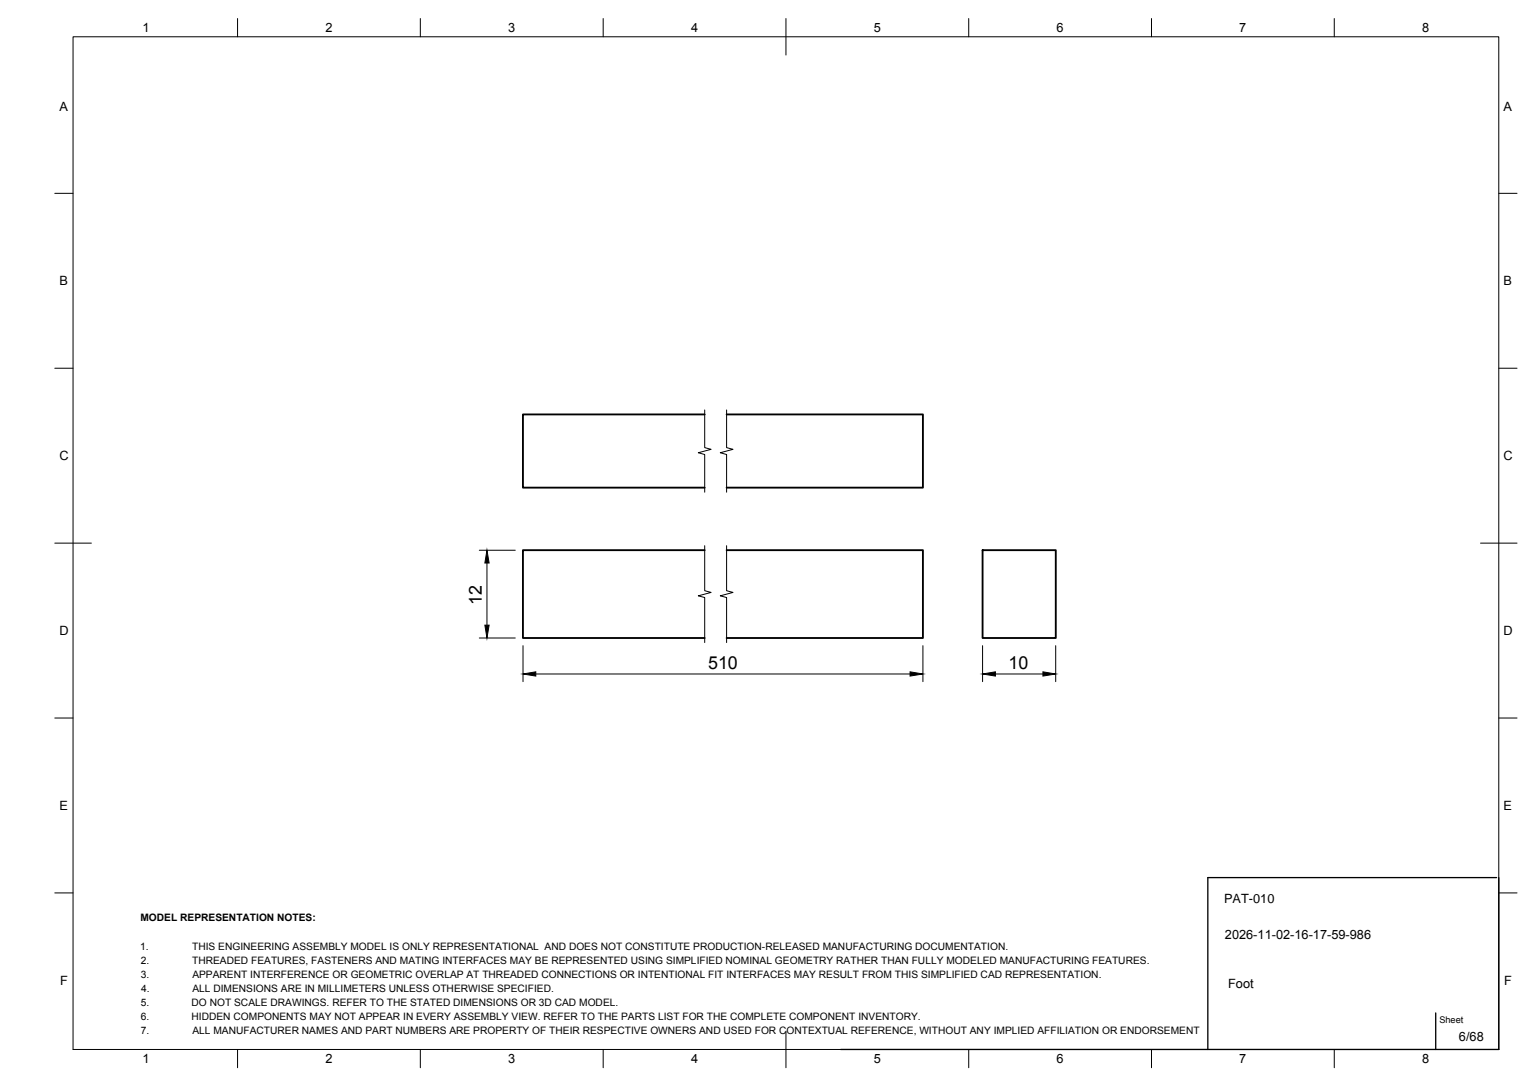
ISO-10303-21;
HEADER;
/* Generated by software containing ST-Developer
 * from STEP Tools, Inc. (www.steptools.com) 
 */

FILE_DESCRIPTION(
/* description */ ('Belt conveyor head drive unit'),
/* implementation_level */ '2;1');

FILE_NAME(
/* name */ 'Foot.step',
/* time_stamp */ '2026-10-28T03:26:19-07:00',
/* author */ (''),
/* organization */ (''),
/* preprocessor_version */ 'ST-DEVELOPER v20.2',
/* originating_system */ 'Autodesk Translation Framework v15.17.0.0',
/* authorisation */ '');

FILE_SCHEMA (('AUTOMOTIVE_DESIGN { 1 0 10303 214 3 1 1 }'));
ENDSEC;

DATA;
#10=MECHANICAL_DESIGN_GEOMETRIC_PRESENTATION_REPRESENTATION('',(#848),#27069);
#710=SHAPE_REPRESENTATION_RELATIONSHIP('SRR','None',#27354,#779);
#779=ADVANCED_BREP_SHAPE_REPRESENTATION('',(#933),#26996);
#848=STYLED_ITEM('',(#27811),#933);
#933=MANIFOLD_SOLID_BREP('Body1',#13713);
#1305=PLANE('',#14664);
#1306=PLANE('',#14665);
#1307=PLANE('',#14666);
#1308=PLANE('',#14667);
#1309=PLANE('',#14668);
#1310=PLANE('',#14669);
#1683=FACE_OUTER_BOUND('',#2503,.T.);
#1684=FACE_OUTER_BOUND('',#2504,.T.);
#1685=FACE_OUTER_BOUND('',#2505,.T.);
#1686=FACE_OUTER_BOUND('',#2506,.T.);
#1687=FACE_OUTER_BOUND('',#2507,.T.);
#1688=FACE_OUTER_BOUND('',#2508,.T.);
#2503=EDGE_LOOP('',(#9174,#9175,#9176,#9177));
#2504=EDGE_LOOP('',(#9178,#9179,#9180,#9181));
#2505=EDGE_LOOP('',(#9182,#9183,#9184,#9185));
#2506=EDGE_LOOP('',(#9186,#9187,#9188,#9189));
#2507=EDGE_LOOP('',(#9190,#9191,#9192,#9193));
#2508=EDGE_LOOP('',(#9194,#9195,#9196,#9197));
#3558=LINE('',#21207,#4350);
#3559=LINE('',#21209,#4351);
#3560=LINE('',#21211,#4352);
#3561=LINE('',#21212,#4353);
#3562=LINE('',#21215,#4354);
#3563=LINE('',#21217,#4355);
#3564=LINE('',#21218,#4356);
#3565=LINE('',#21221,#4357);
#3566=LINE('',#21223,#4358);
#3567=LINE('',#21224,#4359);
#3568=LINE('',#21226,#4360);
#3569=LINE('',#21227,#4361);
#4350=VECTOR('',#16700,1.);
#4351=VECTOR('',#16701,1.);
#4352=VECTOR('',#16702,1.);
#4353=VECTOR('',#16703,1.);
#4354=VECTOR('',#16706,1.);
#4355=VECTOR('',#16707,1.);
#4356=VECTOR('',#16708,1.);
#4357=VECTOR('',#16711,1.);
#4358=VECTOR('',#16712,1.);
#4359=VECTOR('',#16713,1.);
#4360=VECTOR('',#16716,1.);
#4361=VECTOR('',#16717,1.);
#6025=VERTEX_POINT('',#21205);
#6026=VERTEX_POINT('',#21206);
#6027=VERTEX_POINT('',#21208);
#6028=VERTEX_POINT('',#21210);
#6029=VERTEX_POINT('',#21214);
#6030=VERTEX_POINT('',#21216);
#6031=VERTEX_POINT('',#21220);
#6032=VERTEX_POINT('',#21222);
#7279=EDGE_CURVE('',#6025,#6026,#3558,.T.);
#7280=EDGE_CURVE('',#6026,#6027,#3559,.T.);
#7281=EDGE_CURVE('',#6028,#6027,#3560,.T.);
#7282=EDGE_CURVE('',#6025,#6028,#3561,.T.);
#7283=EDGE_CURVE('',#6029,#6025,#3562,.T.);
#7284=EDGE_CURVE('',#6030,#6028,#3563,.T.);
#7285=EDGE_CURVE('',#6029,#6030,#3564,.T.);
#7286=EDGE_CURVE('',#6031,#6029,#3565,.T.);
#7287=EDGE_CURVE('',#6032,#6030,#3566,.T.);
#7288=EDGE_CURVE('',#6031,#6032,#3567,.T.);
#7289=EDGE_CURVE('',#6026,#6031,#3568,.T.);
#7290=EDGE_CURVE('',#6027,#6032,#3569,.T.);
#9174=ORIENTED_EDGE('',*,*,#7279,.T.);
#9175=ORIENTED_EDGE('',*,*,#7280,.T.);
#9176=ORIENTED_EDGE('',*,*,#7281,.F.);
#9177=ORIENTED_EDGE('',*,*,#7282,.F.);
#9178=ORIENTED_EDGE('',*,*,#7283,.T.);
#9179=ORIENTED_EDGE('',*,*,#7282,.T.);
#9180=ORIENTED_EDGE('',*,*,#7284,.F.);
#9181=ORIENTED_EDGE('',*,*,#7285,.F.);
#9182=ORIENTED_EDGE('',*,*,#7286,.T.);
#9183=ORIENTED_EDGE('',*,*,#7285,.T.);
#9184=ORIENTED_EDGE('',*,*,#7287,.F.);
#9185=ORIENTED_EDGE('',*,*,#7288,.F.);
#9186=ORIENTED_EDGE('',*,*,#7289,.T.);
#9187=ORIENTED_EDGE('',*,*,#7288,.T.);
#9188=ORIENTED_EDGE('',*,*,#7290,.F.);
#9189=ORIENTED_EDGE('',*,*,#7280,.F.);
#9190=ORIENTED_EDGE('',*,*,#7290,.T.);
#9191=ORIENTED_EDGE('',*,*,#7287,.T.);
#9192=ORIENTED_EDGE('',*,*,#7284,.T.);
#9193=ORIENTED_EDGE('',*,*,#7281,.T.);
#9194=ORIENTED_EDGE('',*,*,#7289,.F.);
#9195=ORIENTED_EDGE('',*,*,#7279,.F.);
#9196=ORIENTED_EDGE('',*,*,#7283,.F.);
#9197=ORIENTED_EDGE('',*,*,#7286,.F.);
#12962=ADVANCED_FACE('',(#1683),#1305,.T.);
#12963=ADVANCED_FACE('',(#1684),#1306,.T.);
#12964=ADVANCED_FACE('',(#1685),#1307,.T.);
#12965=ADVANCED_FACE('',(#1686),#1308,.T.);
#12966=ADVANCED_FACE('',(#1687),#1309,.T.);
#12967=ADVANCED_FACE('',(#1688),#1310,.F.);
#13713=CLOSED_SHELL('',(#12962,#12963,#12964,#12965,#12966,#12967));
#14663=AXIS2_PLACEMENT_3D('',#21203,#16696,#16697);
#14664=AXIS2_PLACEMENT_3D('',#21204,#16698,#16699);
#14665=AXIS2_PLACEMENT_3D('',#21213,#16704,#16705);
#14666=AXIS2_PLACEMENT_3D('',#21219,#16709,#16710);
#14667=AXIS2_PLACEMENT_3D('',#21225,#16714,#16715);
#14668=AXIS2_PLACEMENT_3D('',#21228,#16718,#16719);
#14669=AXIS2_PLACEMENT_3D('',#21229,#16720,#16721);
#16696=DIRECTION('axis',(0.,0.,1.));
#16697=DIRECTION('refdir',(1.,0.,0.));
#16698=DIRECTION('center_axis',(0.,1.,0.));
#16699=DIRECTION('ref_axis',(-1.,0.,0.));
#16700=DIRECTION('',(-1.,0.,0.));
#16701=DIRECTION('',(0.,0.,1.));
#16702=DIRECTION('',(-1.,0.,0.));
#16703=DIRECTION('',(0.,0.,1.));
#16704=DIRECTION('center_axis',(1.,0.,0.));
#16705=DIRECTION('ref_axis',(0.,1.,0.));
#16706=DIRECTION('',(0.,1.,0.));
#16707=DIRECTION('',(0.,1.,0.));
#16708=DIRECTION('',(0.,0.,1.));
#16709=DIRECTION('center_axis',(0.,-1.,0.));
#16710=DIRECTION('ref_axis',(1.,0.,0.));
#16711=DIRECTION('',(1.,0.,0.));
#16712=DIRECTION('',(1.,0.,0.));
#16713=DIRECTION('',(0.,0.,1.));
#16714=DIRECTION('center_axis',(-1.,0.,0.));
#16715=DIRECTION('ref_axis',(0.,-1.,0.));
#16716=DIRECTION('',(0.,-1.,0.));
#16717=DIRECTION('',(0.,-1.,0.));
#16718=DIRECTION('center_axis',(0.,0.,1.));
#16719=DIRECTION('ref_axis',(1.,0.,0.));
#16720=DIRECTION('center_axis',(0.,0.,1.));
#16721=DIRECTION('ref_axis',(1.,0.,0.));
#21203=CARTESIAN_POINT('',(0.,0.,0.));
#21204=CARTESIAN_POINT('Origin',(-3.,44.5,-2.4));
#21205=CARTESIAN_POINT('',(-3.,44.5,-2.4));
#21206=CARTESIAN_POINT('',(-4.,44.5,-2.4));
#21207=CARTESIAN_POINT('',(-3.,44.5,-2.4));
#21208=CARTESIAN_POINT('',(-4.,44.5,-1.2));
#21209=CARTESIAN_POINT('',(-4.,44.5,-2.4));
#21210=CARTESIAN_POINT('',(-3.,44.5,-1.2));
#21211=CARTESIAN_POINT('',(-3.,44.5,-1.2));
#21212=CARTESIAN_POINT('',(-3.,44.5,-2.4));
#21213=CARTESIAN_POINT('Origin',(-3.,-6.5,-2.4));
#21214=CARTESIAN_POINT('',(-3.,-6.5,-2.4));
#21215=CARTESIAN_POINT('',(-3.,-6.5,-2.4));
#21216=CARTESIAN_POINT('',(-3.,-6.5,-1.2));
#21217=CARTESIAN_POINT('',(-3.,-6.5,-1.2));
#21218=CARTESIAN_POINT('',(-3.,-6.5,-2.4));
#21219=CARTESIAN_POINT('Origin',(-4.,-6.5,-2.4));
#21220=CARTESIAN_POINT('',(-4.,-6.5,-2.4));
#21221=CARTESIAN_POINT('',(-4.,-6.5,-2.4));
#21222=CARTESIAN_POINT('',(-4.,-6.5,-1.2));
#21223=CARTESIAN_POINT('',(-4.,-6.5,-1.2));
#21224=CARTESIAN_POINT('',(-4.,-6.5,-2.4));
#21225=CARTESIAN_POINT('Origin',(-4.,44.5,-2.4));
#21226=CARTESIAN_POINT('',(-4.,44.5,-2.4));
#21227=CARTESIAN_POINT('',(-4.,44.5,-1.2));
#21228=CARTESIAN_POINT('Origin',(-3.5,19.,-1.2));
#21229=CARTESIAN_POINT('Origin',(-3.5,19.,-2.4));
#26919=UNCERTAINTY_MEASURE_WITH_UNIT(LENGTH_MEASURE(0.001),#27070,
'DISTANCE_ACCURACY_VALUE',
'Maximum model space distance between geometric entities at asserted c
onnectivities');
#26992=UNCERTAINTY_MEASURE_WITH_UNIT(LENGTH_MEASURE(0.001),#27070,
'DISTANCE_ACCURACY_VALUE',
'Maximum model space distance between geometric entities at asserted c
onnectivities');
#26996=(
GEOMETRIC_REPRESENTATION_CONTEXT(3)
GLOBAL_UNCERTAINTY_ASSIGNED_CONTEXT((#26919))
GLOBAL_UNIT_ASSIGNED_CONTEXT((#27070,#27072,#27073))
REPRESENTATION_CONTEXT('','3D')
);
#27069=(
GEOMETRIC_REPRESENTATION_CONTEXT(3)
GLOBAL_UNCERTAINTY_ASSIGNED_CONTEXT((#26992))
GLOBAL_UNIT_ASSIGNED_CONTEXT((#27070,#27072,#27073))
REPRESENTATION_CONTEXT('','3D')
);
#27070=(
LENGTH_UNIT()
NAMED_UNIT(*)
SI_UNIT(.CENTI.,.METRE.)
);
#27072=(
NAMED_UNIT(*)
PLANE_ANGLE_UNIT()
SI_UNIT($,.RADIAN.)
);
#27073=(
NAMED_UNIT(*)
SI_UNIT($,.STERADIAN.)
SOLID_ANGLE_UNIT()
);
#27077=SHAPE_DEFINITION_REPRESENTATION(#27153,#27354);
#27153=PRODUCT_DEFINITION_SHAPE('',$,#27431);
#27354=SHAPE_REPRESENTATION('',(#14663),#26996);
#27427=PRODUCT_DEFINITION_CONTEXT('part definition',#27657,'design');
#27431=PRODUCT_DEFINITION('Foot','Foot',#27507,#27427);
#27507=PRODUCT_DEFINITION_FORMATION('',$,#27662);
#27657=APPLICATION_CONTEXT(
'Core Data for Automotive Mechanical Design Process');
#27658=PRODUCT_CONTEXT('part definition',#27657,'mechanical');
#27662=PRODUCT('Foot','Foot','Foot',(#27658));
#27805=COLOUR_RGB('Off White',0.89,0.88,0.83);
#27806=FILL_AREA_STYLE_COLOUR('',#27805);
#27807=FILL_AREA_STYLE('',(#27806));
#27808=SURFACE_STYLE_FILL_AREA(#27807);
#27809=SURFACE_SIDE_STYLE('',(#27808));
#27810=SURFACE_STYLE_USAGE(.BOTH.,#27809);
#27811=PRESENTATION_STYLE_ASSIGNMENT((#27810));
ENDSEC;
END-ISO-10303-21;
